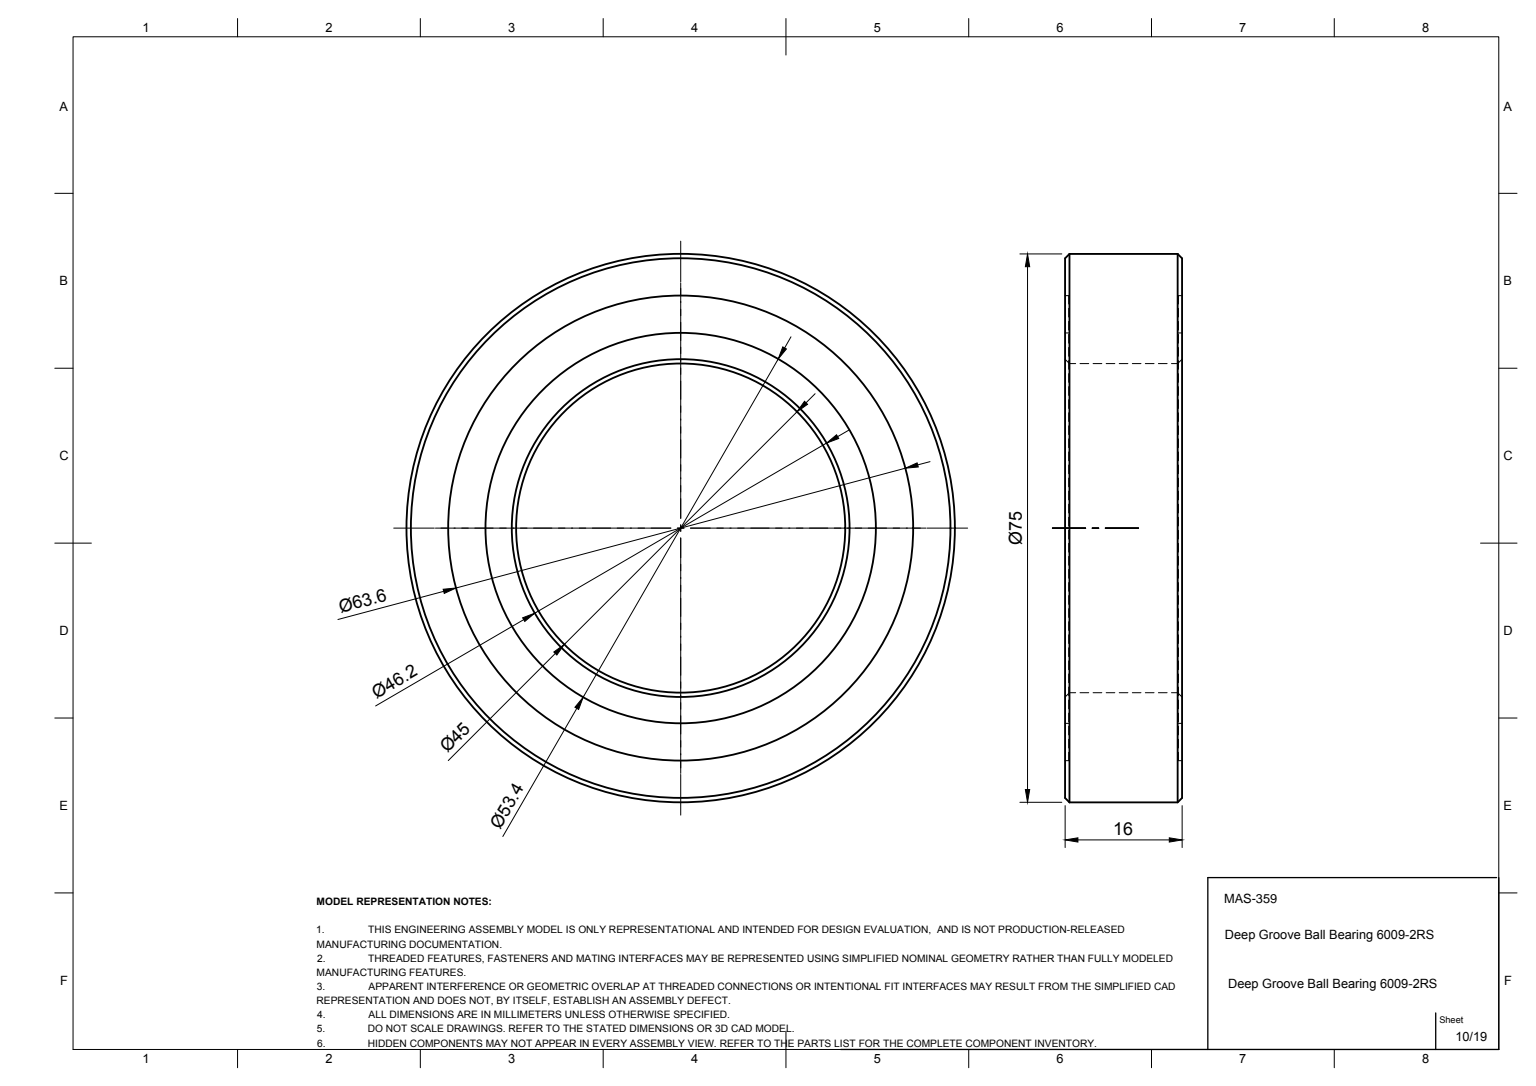
ISO-10303-21;
HEADER;
/* Generated by software containing ST-Developer
 * from STEP Tools, Inc. (www.steptools.com) 
 */

FILE_DESCRIPTION(
/* description */ (''),
/* implementation_level */ '2;1');

FILE_NAME(
/* name */ 'Deep Groove Ball Bearing 6009-2RS.step',
/* time_stamp */ '2026-10-15T14:25:16-07:00',
/* author */ (''),
/* organization */ (''),
/* preprocessor_version */ 'ST-DEVELOPER v20.2',
/* originating_system */ 'Autodesk Translation Framework v15.15.0.0',
/* authorisation */ '');

FILE_SCHEMA (('AUTOMOTIVE_DESIGN { 1 0 10303 214 3 1 1 }'));
ENDSEC;

DATA;
#10=MECHANICAL_DESIGN_GEOMETRIC_PRESENTATION_REPRESENTATION('',(#335),#86429);
#299=SHAPE_REPRESENTATION_RELATIONSHIP('SRR','None',#86514,#317);
#317=ADVANCED_BREP_SHAPE_REPRESENTATION('',(#353),#86423);
#335=STYLED_ITEM('',(#86613),#353);
#353=MANIFOLD_SOLID_BREP('Body1',#15625);
#1327=CONICAL_SURFACE('',#17032,2.28,0.785398163397449);
#1328=CONICAL_SURFACE('',#17044,3.72,0.785398163397449);
#1329=CONICAL_SURFACE('',#17048,3.72,0.785398163397448);
#1330=CONICAL_SURFACE('',#17060,2.28,0.785398163397448);
#1542=CYLINDRICAL_SURFACE('',#17029,2.25);
#1543=CYLINDRICAL_SURFACE('',#17036,2.67);
#1544=CYLINDRICAL_SURFACE('',#17040,3.18);
#1545=CYLINDRICAL_SURFACE('',#17046,3.75);
#1546=CYLINDRICAL_SURFACE('',#17052,3.18);
#1547=CYLINDRICAL_SURFACE('',#17056,2.67);
#1733=FACE_BOUND('',#4130,.T.);
#1734=FACE_BOUND('',#4133,.T.);
#1735=FACE_BOUND('',#4136,.T.);
#1736=FACE_BOUND('',#4141,.T.);
#1737=FACE_BOUND('',#4144,.T.);
#1738=FACE_BOUND('',#4147,.T.);
#2291=CIRCLE('',#17030,2.25);
#2292=CIRCLE('',#17031,2.25);
#2293=CIRCLE('',#17033,2.31);
#2294=CIRCLE('',#17035,2.67);
#2295=CIRCLE('',#17037,2.67);
#2296=CIRCLE('',#17039,3.18);
#2297=CIRCLE('',#17041,3.18);
#2298=CIRCLE('',#17043,3.69);
#2299=CIRCLE('',#17045,3.75);
#2300=CIRCLE('',#17047,3.75);
#2301=CIRCLE('',#17049,3.69);
#2302=CIRCLE('',#17051,3.18);
#2303=CIRCLE('',#17053,3.18);
#2304=CIRCLE('',#17055,2.67);
#2305=CIRCLE('',#17057,2.67);
#2306=CIRCLE('',#17059,2.31);
#3124=FACE_OUTER_BOUND('',#4127,.T.);
#3125=FACE_OUTER_BOUND('',#4128,.T.);
#3126=FACE_OUTER_BOUND('',#4129,.T.);
#3127=FACE_OUTER_BOUND('',#4131,.T.);
#3128=FACE_OUTER_BOUND('',#4132,.T.);
#3129=FACE_OUTER_BOUND('',#4134,.T.);
#3130=FACE_OUTER_BOUND('',#4135,.T.);
#3131=FACE_OUTER_BOUND('',#4137,.T.);
#3132=FACE_OUTER_BOUND('',#4138,.T.);
#3133=FACE_OUTER_BOUND('',#4139,.T.);
#3134=FACE_OUTER_BOUND('',#4140,.T.);
#3135=FACE_OUTER_BOUND('',#4142,.T.);
#3136=FACE_OUTER_BOUND('',#4143,.T.);
#3137=FACE_OUTER_BOUND('',#4145,.T.);
#3138=FACE_OUTER_BOUND('',#4146,.T.);
#3139=FACE_OUTER_BOUND('',#4148,.T.);
#4127=EDGE_LOOP('',(#13627,#13628,#13629,#13630));
#4128=EDGE_LOOP('',(#13631,#13632,#13633,#13634));
#4129=EDGE_LOOP('',(#13635));
#4130=EDGE_LOOP('',(#13636));
#4131=EDGE_LOOP('',(#13637,#13638,#13639,#13640));
#4132=EDGE_LOOP('',(#13641));
#4133=EDGE_LOOP('',(#13642));
#4134=EDGE_LOOP('',(#13643,#13644,#13645,#13646));
#4135=EDGE_LOOP('',(#13647));
#4136=EDGE_LOOP('',(#13648));
#4137=EDGE_LOOP('',(#13649,#13650,#13651,#13652));
#4138=EDGE_LOOP('',(#13653,#13654,#13655,#13656));
#4139=EDGE_LOOP('',(#13657,#13658,#13659,#13660));
#4140=EDGE_LOOP('',(#13661));
#4141=EDGE_LOOP('',(#13662));
#4142=EDGE_LOOP('',(#13663,#13664,#13665,#13666));
#4143=EDGE_LOOP('',(#13667));
#4144=EDGE_LOOP('',(#13668));
#4145=EDGE_LOOP('',(#13669,#13670,#13671,#13672));
#4146=EDGE_LOOP('',(#13673));
#4147=EDGE_LOOP('',(#13674));
#4148=EDGE_LOOP('',(#13675,#13676,#13677,#13678));
#5031=LINE('',#66455,#5891);
#5032=LINE('',#66459,#5892);
#5033=LINE('',#66467,#5893);
#5034=LINE('',#66474,#5894);
#5035=LINE('',#66481,#5895);
#5036=LINE('',#66485,#5896);
#5037=LINE('',#66488,#5897);
#5038=LINE('',#66496,#5898);
#5039=LINE('',#66503,#5899);
#5040=LINE('',#66508,#5900);
#5891=VECTOR('',#20438,2.25);
#5892=VECTOR('',#20443,2.28);
#5893=VECTOR('',#20454,2.67);
#5894=VECTOR('',#20463,3.18);
#5895=VECTOR('',#20472,3.72);
#5896=VECTOR('',#20477,3.75);
#5897=VECTOR('',#20480,3.72);
#5898=VECTOR('',#20491,3.18);
#5899=VECTOR('',#20500,2.67);
#5900=VECTOR('',#20507,2.28);
#7239=VERTEX_POINT('',#66452);
#7240=VERTEX_POINT('',#66454);
#7241=VERTEX_POINT('',#66458);
#7242=VERTEX_POINT('',#66462);
#7243=VERTEX_POINT('',#66465);
#7244=VERTEX_POINT('',#66469);
#7245=VERTEX_POINT('',#66472);
#7246=VERTEX_POINT('',#66476);
#7247=VERTEX_POINT('',#66479);
#7248=VERTEX_POINT('',#66483);
#7249=VERTEX_POINT('',#66487);
#7250=VERTEX_POINT('',#66491);
#7251=VERTEX_POINT('',#66494);
#7252=VERTEX_POINT('',#66498);
#7253=VERTEX_POINT('',#66501);
#7254=VERTEX_POINT('',#66505);
#9435=EDGE_CURVE('',#7239,#7239,#2291,.T.);
#9436=EDGE_CURVE('',#7239,#7240,#5031,.T.);
#9437=EDGE_CURVE('',#7240,#7240,#2292,.T.);
#9438=EDGE_CURVE('',#7239,#7241,#5032,.T.);
#9439=EDGE_CURVE('',#7241,#7241,#2293,.T.);
#9440=EDGE_CURVE('',#7242,#7242,#2294,.T.);
#9441=EDGE_CURVE('',#7243,#7243,#2295,.T.);
#9442=EDGE_CURVE('',#7243,#7242,#5033,.T.);
#9443=EDGE_CURVE('',#7244,#7244,#2296,.T.);
#9444=EDGE_CURVE('',#7245,#7245,#2297,.T.);
#9445=EDGE_CURVE('',#7245,#7244,#5034,.T.);
#9446=EDGE_CURVE('',#7246,#7246,#2298,.T.);
#9447=EDGE_CURVE('',#7247,#7247,#2299,.T.);
#9448=EDGE_CURVE('',#7247,#7246,#5035,.T.);
#9449=EDGE_CURVE('',#7248,#7248,#2300,.T.);
#9450=EDGE_CURVE('',#7248,#7247,#5036,.T.);
#9451=EDGE_CURVE('',#7248,#7249,#5037,.T.);
#9452=EDGE_CURVE('',#7249,#7249,#2301,.T.);
#9453=EDGE_CURVE('',#7250,#7250,#2302,.T.);
#9454=EDGE_CURVE('',#7251,#7251,#2303,.T.);
#9455=EDGE_CURVE('',#7251,#7250,#5038,.T.);
#9456=EDGE_CURVE('',#7252,#7252,#2304,.T.);
#9457=EDGE_CURVE('',#7253,#7253,#2305,.T.);
#9458=EDGE_CURVE('',#7253,#7252,#5039,.T.);
#9459=EDGE_CURVE('',#7254,#7254,#2306,.T.);
#9460=EDGE_CURVE('',#7240,#7254,#5040,.T.);
#13627=ORIENTED_EDGE('',*,*,#9435,.F.);
#13628=ORIENTED_EDGE('',*,*,#9436,.T.);
#13629=ORIENTED_EDGE('',*,*,#9437,.T.);
#13630=ORIENTED_EDGE('',*,*,#9436,.F.);
#13631=ORIENTED_EDGE('',*,*,#9435,.T.);
#13632=ORIENTED_EDGE('',*,*,#9438,.T.);
#13633=ORIENTED_EDGE('',*,*,#9439,.F.);
#13634=ORIENTED_EDGE('',*,*,#9438,.F.);
#13635=ORIENTED_EDGE('',*,*,#9440,.F.);
#13636=ORIENTED_EDGE('',*,*,#9439,.T.);
#13637=ORIENTED_EDGE('',*,*,#9441,.F.);
#13638=ORIENTED_EDGE('',*,*,#9442,.T.);
#13639=ORIENTED_EDGE('',*,*,#9440,.T.);
#13640=ORIENTED_EDGE('',*,*,#9442,.F.);
#13641=ORIENTED_EDGE('',*,*,#9443,.F.);
#13642=ORIENTED_EDGE('',*,*,#9441,.T.);
#13643=ORIENTED_EDGE('',*,*,#9444,.F.);
#13644=ORIENTED_EDGE('',*,*,#9445,.T.);
#13645=ORIENTED_EDGE('',*,*,#9443,.T.);
#13646=ORIENTED_EDGE('',*,*,#9445,.F.);
#13647=ORIENTED_EDGE('',*,*,#9446,.F.);
#13648=ORIENTED_EDGE('',*,*,#9444,.T.);
#13649=ORIENTED_EDGE('',*,*,#9447,.F.);
#13650=ORIENTED_EDGE('',*,*,#9448,.T.);
#13651=ORIENTED_EDGE('',*,*,#9446,.T.);
#13652=ORIENTED_EDGE('',*,*,#9448,.F.);
#13653=ORIENTED_EDGE('',*,*,#9449,.F.);
#13654=ORIENTED_EDGE('',*,*,#9450,.T.);
#13655=ORIENTED_EDGE('',*,*,#9447,.T.);
#13656=ORIENTED_EDGE('',*,*,#9450,.F.);
#13657=ORIENTED_EDGE('',*,*,#9449,.T.);
#13658=ORIENTED_EDGE('',*,*,#9451,.T.);
#13659=ORIENTED_EDGE('',*,*,#9452,.F.);
#13660=ORIENTED_EDGE('',*,*,#9451,.F.);
#13661=ORIENTED_EDGE('',*,*,#9452,.T.);
#13662=ORIENTED_EDGE('',*,*,#9453,.F.);
#13663=ORIENTED_EDGE('',*,*,#9454,.F.);
#13664=ORIENTED_EDGE('',*,*,#9455,.T.);
#13665=ORIENTED_EDGE('',*,*,#9453,.T.);
#13666=ORIENTED_EDGE('',*,*,#9455,.F.);
#13667=ORIENTED_EDGE('',*,*,#9454,.T.);
#13668=ORIENTED_EDGE('',*,*,#9456,.F.);
#13669=ORIENTED_EDGE('',*,*,#9457,.F.);
#13670=ORIENTED_EDGE('',*,*,#9458,.T.);
#13671=ORIENTED_EDGE('',*,*,#9456,.T.);
#13672=ORIENTED_EDGE('',*,*,#9458,.F.);
#13673=ORIENTED_EDGE('',*,*,#9457,.T.);
#13674=ORIENTED_EDGE('',*,*,#9459,.F.);
#13675=ORIENTED_EDGE('',*,*,#9437,.F.);
#13676=ORIENTED_EDGE('',*,*,#9460,.T.);
#13677=ORIENTED_EDGE('',*,*,#9459,.T.);
#13678=ORIENTED_EDGE('',*,*,#9460,.F.);
#14700=PLANE('',#17034);
#14701=PLANE('',#17038);
#14702=PLANE('',#17042);
#14703=PLANE('',#17050);
#14704=PLANE('',#17054);
#14705=PLANE('',#17058);
#15480=ADVANCED_FACE('',(#3124),#1542,.F.);
#15481=ADVANCED_FACE('',(#3125),#1327,.F.);
#15482=ADVANCED_FACE('',(#3126,#1733),#14700,.T.);
#15483=ADVANCED_FACE('',(#3127),#1543,.T.);
#15484=ADVANCED_FACE('',(#3128,#1734),#14701,.T.);
#15485=ADVANCED_FACE('',(#3129),#1544,.F.);
#15486=ADVANCED_FACE('',(#3130,#1735),#14702,.T.);
#15487=ADVANCED_FACE('',(#3131),#1328,.T.);
#15488=ADVANCED_FACE('',(#3132),#1545,.T.);
#15489=ADVANCED_FACE('',(#3133),#1329,.T.);
#15490=ADVANCED_FACE('',(#3134,#1736),#14703,.T.);
#15491=ADVANCED_FACE('',(#3135),#1546,.F.);
#15492=ADVANCED_FACE('',(#3136,#1737),#14704,.T.);
#15493=ADVANCED_FACE('',(#3137),#1547,.T.);
#15494=ADVANCED_FACE('',(#3138,#1738),#14705,.T.);
#15495=ADVANCED_FACE('',(#3139),#1330,.F.);
#15625=CLOSED_SHELL('',(#15480,#15481,#15482,#15483,#15484,#15485,#15486,
#15487,#15488,#15489,#15490,#15491,#15492,#15493,#15494,#15495));
#17028=AXIS2_PLACEMENT_3D('',#66450,#20432,#20433);
#17029=AXIS2_PLACEMENT_3D('',#66451,#20434,#20435);
#17030=AXIS2_PLACEMENT_3D('',#66453,#20436,#20437);
#17031=AXIS2_PLACEMENT_3D('',#66456,#20439,#20440);
#17032=AXIS2_PLACEMENT_3D('',#66457,#20441,#20442);
#17033=AXIS2_PLACEMENT_3D('',#66460,#20444,#20445);
#17034=AXIS2_PLACEMENT_3D('',#66461,#20446,#20447);
#17035=AXIS2_PLACEMENT_3D('',#66463,#20448,#20449);
#17036=AXIS2_PLACEMENT_3D('',#66464,#20450,#20451);
#17037=AXIS2_PLACEMENT_3D('',#66466,#20452,#20453);
#17038=AXIS2_PLACEMENT_3D('',#66468,#20455,#20456);
#17039=AXIS2_PLACEMENT_3D('',#66470,#20457,#20458);
#17040=AXIS2_PLACEMENT_3D('',#66471,#20459,#20460);
#17041=AXIS2_PLACEMENT_3D('',#66473,#20461,#20462);
#17042=AXIS2_PLACEMENT_3D('',#66475,#20464,#20465);
#17043=AXIS2_PLACEMENT_3D('',#66477,#20466,#20467);
#17044=AXIS2_PLACEMENT_3D('',#66478,#20468,#20469);
#17045=AXIS2_PLACEMENT_3D('',#66480,#20470,#20471);
#17046=AXIS2_PLACEMENT_3D('',#66482,#20473,#20474);
#17047=AXIS2_PLACEMENT_3D('',#66484,#20475,#20476);
#17048=AXIS2_PLACEMENT_3D('',#66486,#20478,#20479);
#17049=AXIS2_PLACEMENT_3D('',#66489,#20481,#20482);
#17050=AXIS2_PLACEMENT_3D('',#66490,#20483,#20484);
#17051=AXIS2_PLACEMENT_3D('',#66492,#20485,#20486);
#17052=AXIS2_PLACEMENT_3D('',#66493,#20487,#20488);
#17053=AXIS2_PLACEMENT_3D('',#66495,#20489,#20490);
#17054=AXIS2_PLACEMENT_3D('',#66497,#20492,#20493);
#17055=AXIS2_PLACEMENT_3D('',#66499,#20494,#20495);
#17056=AXIS2_PLACEMENT_3D('',#66500,#20496,#20497);
#17057=AXIS2_PLACEMENT_3D('',#66502,#20498,#20499);
#17058=AXIS2_PLACEMENT_3D('',#66504,#20501,#20502);
#17059=AXIS2_PLACEMENT_3D('',#66506,#20503,#20504);
#17060=AXIS2_PLACEMENT_3D('',#66507,#20505,#20506);
#20432=DIRECTION('axis',(0.,0.,1.));
#20433=DIRECTION('refdir',(1.,0.,0.));
#20434=DIRECTION('center_axis',(0.,0.,1.));
#20435=DIRECTION('ref_axis',(1.,0.,0.));
#20436=DIRECTION('center_axis',(0.,0.,1.));
#20437=DIRECTION('ref_axis',(1.,0.,0.));
#20438=DIRECTION('',(0.,0.,1.));
#20439=DIRECTION('center_axis',(0.,0.,1.));
#20440=DIRECTION('ref_axis',(1.,0.,0.));
#20441=DIRECTION('center_axis',(0.,0.,-1.));
#20442=DIRECTION('ref_axis',(1.,0.,0.));
#20443=DIRECTION('',(-0.707106781186548,8.65956056235494E-17,-0.707106781186547));
#20444=DIRECTION('center_axis',(0.,0.,1.));
#20445=DIRECTION('ref_axis',(1.,0.,0.));
#20446=DIRECTION('center_axis',(0.,0.,-1.));
#20447=DIRECTION('ref_axis',(-1.,0.,0.));
#20448=DIRECTION('center_axis',(0.,0.,1.));
#20449=DIRECTION('ref_axis',(1.,0.,0.));
#20450=DIRECTION('center_axis',(0.,0.,1.));
#20451=DIRECTION('ref_axis',(1.,0.,0.));
#20452=DIRECTION('center_axis',(0.,0.,1.));
#20453=DIRECTION('ref_axis',(1.,0.,0.));
#20454=DIRECTION('',(0.,0.,-1.));
#20455=DIRECTION('center_axis',(0.,0.,-1.));
#20456=DIRECTION('ref_axis',(-1.,0.,0.));
#20457=DIRECTION('center_axis',(0.,0.,1.));
#20458=DIRECTION('ref_axis',(1.,0.,0.));
#20459=DIRECTION('center_axis',(0.,0.,1.));
#20460=DIRECTION('ref_axis',(1.,0.,0.));
#20461=DIRECTION('center_axis',(0.,0.,1.));
#20462=DIRECTION('ref_axis',(1.,0.,0.));
#20463=DIRECTION('',(0.,0.,1.));
#20464=DIRECTION('center_axis',(0.,0.,-1.));
#20465=DIRECTION('ref_axis',(-1.,0.,0.));
#20466=DIRECTION('center_axis',(0.,0.,1.));
#20467=DIRECTION('ref_axis',(1.,0.,0.));
#20468=DIRECTION('center_axis',(0.,0.,1.));
#20469=DIRECTION('ref_axis',(1.,0.,0.));
#20470=DIRECTION('center_axis',(0.,0.,1.));
#20471=DIRECTION('ref_axis',(1.,0.,0.));
#20472=DIRECTION('',(0.707106781186548,8.65956056235494E-17,-0.707106781186547));
#20473=DIRECTION('center_axis',(0.,0.,1.));
#20474=DIRECTION('ref_axis',(1.,0.,0.));
#20475=DIRECTION('center_axis',(0.,0.,1.));
#20476=DIRECTION('ref_axis',(1.,0.,0.));
#20477=DIRECTION('',(0.,0.,-1.));
#20478=DIRECTION('center_axis',(0.,0.,-1.));
#20479=DIRECTION('ref_axis',(1.,0.,0.));
#20480=DIRECTION('',(0.707106781186547,-8.65956056235493E-17,0.707106781186548));
#20481=DIRECTION('center_axis',(0.,0.,1.));
#20482=DIRECTION('ref_axis',(1.,0.,0.));
#20483=DIRECTION('center_axis',(0.,0.,1.));
#20484=DIRECTION('ref_axis',(1.,0.,0.));
#20485=DIRECTION('center_axis',(0.,0.,1.));
#20486=DIRECTION('ref_axis',(1.,0.,0.));
#20487=DIRECTION('center_axis',(0.,0.,1.));
#20488=DIRECTION('ref_axis',(1.,0.,0.));
#20489=DIRECTION('center_axis',(0.,0.,1.));
#20490=DIRECTION('ref_axis',(1.,0.,0.));
#20491=DIRECTION('',(0.,0.,1.));
#20492=DIRECTION('center_axis',(0.,0.,1.));
#20493=DIRECTION('ref_axis',(1.,0.,0.));
#20494=DIRECTION('center_axis',(0.,0.,1.));
#20495=DIRECTION('ref_axis',(1.,0.,0.));
#20496=DIRECTION('center_axis',(0.,0.,1.));
#20497=DIRECTION('ref_axis',(1.,0.,0.));
#20498=DIRECTION('center_axis',(0.,0.,1.));
#20499=DIRECTION('ref_axis',(1.,0.,0.));
#20500=DIRECTION('',(0.,0.,-1.));
#20501=DIRECTION('center_axis',(0.,0.,1.));
#20502=DIRECTION('ref_axis',(1.,0.,0.));
#20503=DIRECTION('center_axis',(0.,0.,1.));
#20504=DIRECTION('ref_axis',(1.,0.,0.));
#20505=DIRECTION('center_axis',(0.,0.,1.));
#20506=DIRECTION('ref_axis',(1.,0.,0.));
#20507=DIRECTION('',(-0.707106781186547,-8.65956056235493E-17,0.707106781186548));
#66450=CARTESIAN_POINT('',(0.,0.,0.));
#66451=CARTESIAN_POINT('Origin',(0.,0.,0.8));
#66452=CARTESIAN_POINT('',(-2.25,-2.75545529808154E-16,0.0600000000000001));
#66453=CARTESIAN_POINT('Origin',(0.,0.,0.0600000000000001));
#66454=CARTESIAN_POINT('',(-2.25,-2.75545529808154E-16,1.54));
#66455=CARTESIAN_POINT('',(-2.25,-2.75545529808154E-16,0.8));
#66456=CARTESIAN_POINT('Origin',(0.,0.,1.54));
#66457=CARTESIAN_POINT('Origin',(0.,0.,0.03));
#66458=CARTESIAN_POINT('',(-2.31,-2.82893410603039E-16,1.28369537222284E-16));
#66459=CARTESIAN_POINT('',(-2.28,2.79219470205597E-16,0.03));
#66460=CARTESIAN_POINT('Origin',(0.,0.,0.));
#66461=CARTESIAN_POINT('Origin',(2.67,0.,0.));
#66462=CARTESIAN_POINT('',(-2.67,-3.26980695372343E-16,0.));
#66463=CARTESIAN_POINT('Origin',(0.,0.,0.));
#66464=CARTESIAN_POINT('Origin',(0.,0.,0.0249999999999999));
#66465=CARTESIAN_POINT('',(-2.67,-3.26980695372343E-16,0.05));
#66466=CARTESIAN_POINT('Origin',(0.,0.,0.05));
#66467=CARTESIAN_POINT('',(-2.67,-3.26980695372343E-16,0.0249999999999999));
#66468=CARTESIAN_POINT('Origin',(3.18,0.,0.05));
#66469=CARTESIAN_POINT('',(-3.18,-3.89437682128858E-16,0.05));
#66470=CARTESIAN_POINT('Origin',(0.,0.,0.05));
#66471=CARTESIAN_POINT('Origin',(0.,0.,0.0249999999999999));
#66472=CARTESIAN_POINT('',(-3.18,-3.89437682128858E-16,-3.46944695195361E-18));
#66473=CARTESIAN_POINT('Origin',(0.,0.,0.));
#66474=CARTESIAN_POINT('',(-3.18,-3.89437682128858E-16,0.0249999999999999));
#66475=CARTESIAN_POINT('Origin',(3.69,0.,0.));
#66476=CARTESIAN_POINT('',(-3.69,-4.51894668885373E-16,1.28369537222284E-16));
#66477=CARTESIAN_POINT('Origin',(0.,0.,0.));
#66478=CARTESIAN_POINT('Origin',(0.,0.,0.03));
#66479=CARTESIAN_POINT('',(-3.75,-4.59242549680257E-16,0.0600000000000002));
#66480=CARTESIAN_POINT('Origin',(0.,0.,0.0600000000000001));
#66481=CARTESIAN_POINT('',(-3.72,-4.55568609282815E-16,0.03));
#66482=CARTESIAN_POINT('Origin',(0.,0.,0.8));
#66483=CARTESIAN_POINT('',(-3.75,-4.59242549680257E-16,1.54));
#66484=CARTESIAN_POINT('Origin',(0.,0.,1.54));
#66485=CARTESIAN_POINT('',(-3.75,-4.59242549680257E-16,0.8));
#66486=CARTESIAN_POINT('Origin',(0.,0.,1.57));
#66487=CARTESIAN_POINT('',(-3.69,-4.51894668885373E-16,1.6));
#66488=CARTESIAN_POINT('',(-3.72,4.55568609282815E-16,1.57));
#66489=CARTESIAN_POINT('Origin',(0.,0.,1.6));
#66490=CARTESIAN_POINT('Origin',(3.18,0.,1.6));
#66491=CARTESIAN_POINT('',(-3.18,-3.89437682128858E-16,1.6));
#66492=CARTESIAN_POINT('Origin',(0.,0.,1.6));
#66493=CARTESIAN_POINT('Origin',(0.,0.,1.575));
#66494=CARTESIAN_POINT('',(-3.18,-3.89437682128858E-16,1.55));
#66495=CARTESIAN_POINT('Origin',(0.,0.,1.55));
#66496=CARTESIAN_POINT('',(-3.18,-3.89437682128858E-16,1.575));
#66497=CARTESIAN_POINT('Origin',(2.67,0.,1.55));
#66498=CARTESIAN_POINT('',(-2.67,-3.26980695372343E-16,1.55));
#66499=CARTESIAN_POINT('Origin',(0.,0.,1.55));
#66500=CARTESIAN_POINT('Origin',(0.,0.,1.575));
#66501=CARTESIAN_POINT('',(-2.67,-3.26980695372343E-16,1.6));
#66502=CARTESIAN_POINT('Origin',(0.,0.,1.6));
#66503=CARTESIAN_POINT('',(-2.67,-3.26980695372343E-16,1.575));
#66504=CARTESIAN_POINT('Origin',(2.31,0.,1.6));
#66505=CARTESIAN_POINT('',(-2.31,-2.82893410603039E-16,1.6));
#66506=CARTESIAN_POINT('Origin',(0.,0.,1.6));
#66507=CARTESIAN_POINT('Origin',(0.,0.,1.57));
#66508=CARTESIAN_POINT('',(-2.28,-2.79219470205597E-16,1.57));
#86403=UNCERTAINTY_MEASURE_WITH_UNIT(LENGTH_MEASURE(0.001),#86430,
'DISTANCE_ACCURACY_VALUE',
'Maximum model space distance between geometric entities at asserted c
onnectivities');
#86409=UNCERTAINTY_MEASURE_WITH_UNIT(LENGTH_MEASURE(0.001),#86430,
'DISTANCE_ACCURACY_VALUE',
'Maximum model space distance between geometric entities at asserted c
onnectivities');
#86423=(
GEOMETRIC_REPRESENTATION_CONTEXT(3)
GLOBAL_UNCERTAINTY_ASSIGNED_CONTEXT((#86403))
GLOBAL_UNIT_ASSIGNED_CONTEXT((#86430,#86432,#86433))
REPRESENTATION_CONTEXT('','3D')
);
#86429=(
GEOMETRIC_REPRESENTATION_CONTEXT(3)
GLOBAL_UNCERTAINTY_ASSIGNED_CONTEXT((#86409))
GLOBAL_UNIT_ASSIGNED_CONTEXT((#86430,#86432,#86433))
REPRESENTATION_CONTEXT('','3D')
);
#86430=(
LENGTH_UNIT()
NAMED_UNIT(*)
SI_UNIT(.CENTI.,.METRE.)
);
#86432=(
NAMED_UNIT(*)
PLANE_ANGLE_UNIT()
SI_UNIT($,.RADIAN.)
);
#86433=(
NAMED_UNIT(*)
SI_UNIT($,.STERADIAN.)
SOLID_ANGLE_UNIT()
);
#86447=SHAPE_DEFINITION_REPRESENTATION(#86466,#86514);
#86466=PRODUCT_DEFINITION_SHAPE('',$,#86534);
#86514=SHAPE_REPRESENTATION('',(#17028),#86423);
#86520=PRODUCT_DEFINITION_CONTEXT('part definition',#86579,'design');
#86534=PRODUCT_DEFINITION('Deep Groove Ball Bearing 6009-2RS',
'Deep Groove Ball Bearing 6009-2RS',#86553,#86520);
#86553=PRODUCT_DEFINITION_FORMATION('',$,#86594);
#86579=APPLICATION_CONTEXT(
'Core Data for Automotive Mechanical Design Process');
#86580=PRODUCT_CONTEXT('part definition',#86579,'mechanical');
#86594=PRODUCT('Deep Groove Ball Bearing 6009-2RS',
'Deep Groove Ball Bearing 6009-2RS',$,(#86580));
#86613=PRESENTATION_STYLE_ASSIGNMENT((#86631));
#86631=SURFACE_STYLE_USAGE(.BOTH.,#86649);
#86649=SURFACE_SIDE_STYLE('',(#86667));
#86667=SURFACE_STYLE_FILL_AREA(#86685);
#86685=FILL_AREA_STYLE('Opaque(210,213,218)',(#86703));
#86703=FILL_AREA_STYLE_COLOUR('Opaque(210,213,218)',#86721);
#86721=COLOUR_RGB('Opaque(210,213,218)', 0.09019608, 0.27058824, 0.51372549);
ENDSEC;
END-ISO-10303-21;
